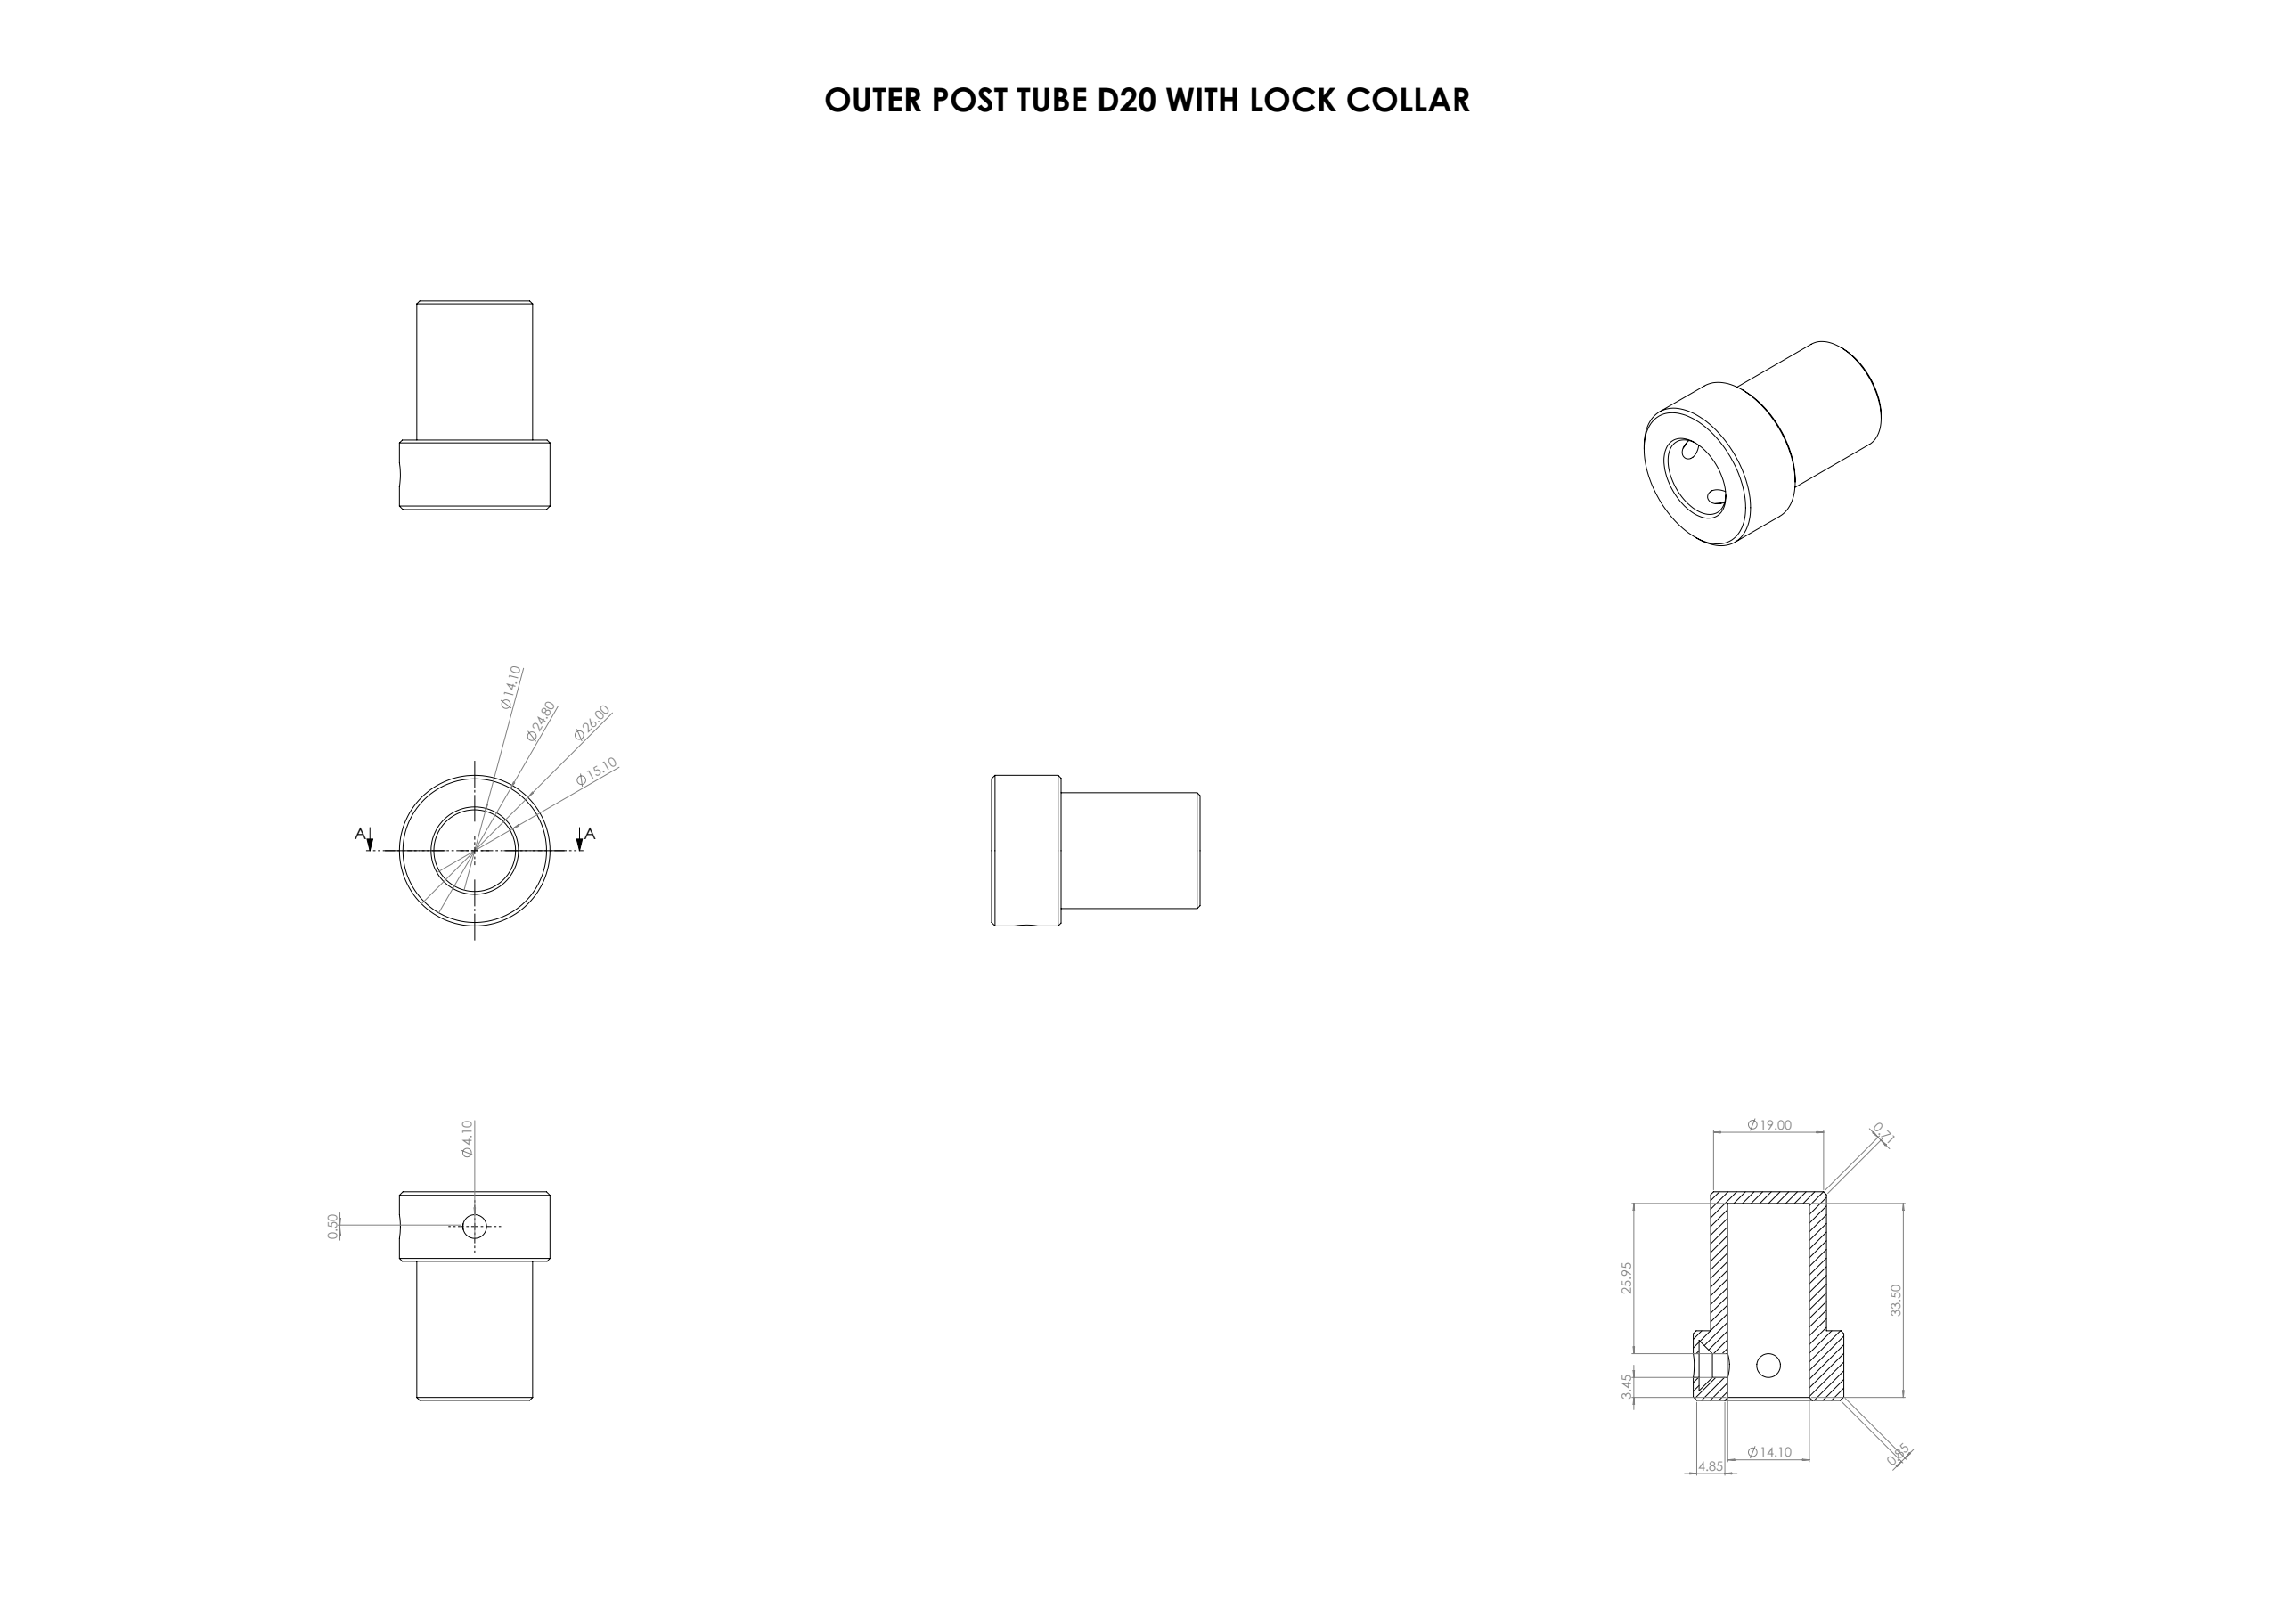
ISO-10303-21;
HEADER;
/* Generated by software containing ST-Developer
 * from STEP Tools, Inc. (www.steptools.com) 
 */

FILE_DESCRIPTION(
/* description */ (''),
/* implementation_level */ '2;1');

FILE_NAME(
/* name */ 
'02_Outer_Post_Tube_D20_with_Lock_Collar.step',
/* time_stamp */ '2026-10-20T10:06:23-07:00',
/* author */ (''),
/* organization */ (''),
/* preprocessor_version */ 'ST-DEVELOPER v20.2',
/* originating_system */ 'Autodesk Translation Framework v15.15.0.0',
/* authorisation */ '');

FILE_SCHEMA (('AUTOMOTIVE_DESIGN { 1 0 10303 214 3 1 1 }'));
ENDSEC;

DATA;
#10=MECHANICAL_DESIGN_GEOMETRIC_PRESENTATION_REPRESENTATION('',(#461),#38611);
#433=SHAPE_REPRESENTATION_RELATIONSHIP('SRR','None',#38669,#447);
#447=ADVANCED_BREP_SHAPE_REPRESENTATION('',(#475),#38598);
#461=STYLED_ITEM('',(#38871),#475);
#475=MANIFOLD_SOLID_BREP('Tube',#16235);
#516=B_SPLINE_CURVE_WITH_KNOTS('',3,(#22682,#22683,#22684,#22685,#22686,
#22687,#22688,#22689,#22690,#22691),.UNSPECIFIED.,.F.,.F.,(4,2,2,2,4),(0.024631319172959,
0.0777176003976506,0.155435200795301,0.233132476857833,0.310829752920366),
 .UNSPECIFIED.);
#517=B_SPLINE_CURVE_WITH_KNOTS('',3,(#22695,#22696,#22697,#22698,#22699,
#22700,#22701,#22702,#22703,#22704),.UNSPECIFIED.,.F.,.F.,(4,2,2,2,4),(0.932489258761097,
1.01018653482363,1.08788381088616,1.16560141128381,1.2186876925085),
 .UNSPECIFIED.);
#518=B_SPLINE_CURVE_WITH_KNOTS('',3,(#22707,#22708,#22709,#22710,#22711,
#22712,#22713,#22714,#22715,#22716),.UNSPECIFIED.,.F.,.F.,(4,2,2,2,4),(0.64629082501369,
0.699377106238382,0.777094706636032,0.854791982698564,0.932489258761097),
 .UNSPECIFIED.);
#519=B_SPLINE_CURVE_WITH_KNOTS('',3,(#22719,#22720,#22721,#22722,#22723,
#22724,#22725,#22726,#22727,#22728),.UNSPECIFIED.,.F.,.F.,(4,2,2,2,4),(0.310829752920366,
0.388527028982898,0.46622430504543,0.54394190544308,0.597028186667772),
 .UNSPECIFIED.);
#520=B_SPLINE_CURVE_WITH_KNOTS('',3,(#22741,#22742,#22743,#22744,#22745,
#22746,#22747,#22748,#22749,#22750,#22751,#22752,#22753,#22754,#22755,#22756,
#22757,#22758,#22759,#22760,#22761,#22762,#22763,#22764,#22765,#22766),
 .UNSPECIFIED.,.F.,.F.,(4,2,2,2,2,2,2,2,2,2,2,2,4),(0.,0.0773604855652864,
0.154720971130573,0.232079805418848,0.309438639707124,0.3867974739954,0.464156308283676,
0.541516793848962,0.618877279414249,0.696237764979535,0.773598250544821,
0.850957084833097,0.928315919121373),.UNSPECIFIED.);
#521=B_SPLINE_CURVE_WITH_KNOTS('',3,(#22767,#22768,#22769,#22770,#22771,
#22772,#22773,#22774,#22775,#22776),.UNSPECIFIED.,.F.,.F.,(4,2,2,2,4),(0.928315919121373,
1.00567475340965,1.08303358769792,1.16039407326321,1.2377545588285),
 .UNSPECIFIED.);
#522=B_SPLINE_CURVE_WITH_KNOTS('',3,(#22786,#22787,#22788,#22789,#22790,
#22791,#22792,#22793,#22794,#22795),.UNSPECIFIED.,.F.,.F.,(4,2,2,2,4),(0.,
0.0773604855652864,0.154720971130573,0.232079805418848,0.309438639707124),
 .UNSPECIFIED.);
#523=B_SPLINE_CURVE_WITH_KNOTS('',3,(#22797,#22798,#22799,#22800,#22801,
#22802,#22803,#22804,#22805,#22806),.UNSPECIFIED.,.F.,.F.,(4,2,2,2,4),(0.928315919121373,
1.00567475340965,1.08303358769792,1.16039407326321,1.2377545588285),
 .UNSPECIFIED.);
#524=B_SPLINE_CURVE_WITH_KNOTS('',3,(#22807,#22808,#22809,#22810,#22811,
#22812,#22813,#22814,#22815,#22816,#22817,#22818,#22819,#22820,#22821,#22822,
#22823,#22824),.UNSPECIFIED.,.F.,.F.,(4,2,2,2,2,2,2,2,4),(0.309438639707124,
0.3867974739954,0.464156308283676,0.541516793848962,0.618877279414249,0.696237764979535,
0.773598250544821,0.850957084833097,0.928315919121373),.UNSPECIFIED.);
#525=B_SPLINE_CURVE_WITH_KNOTS('',3,(#22834,#22835,#22836,#22837,#22838,
#22839,#22840,#22841,#22842,#22843),.UNSPECIFIED.,.F.,.F.,(4,2,2,2,4),(0.0246313191729586,
0.0777176003976506,0.155435200795301,0.233132476857833,0.310829752920366),
 .UNSPECIFIED.);
#526=B_SPLINE_CURVE_WITH_KNOTS('',3,(#22846,#22847,#22848,#22849,#22850,
#22851,#22852,#22853,#22854,#22855,#22856,#22857,#22858,#22859,#22860,#22861,
#22862,#22863),.UNSPECIFIED.,.F.,.F.,(4,2,2,2,2,2,2,2,4),(0.64629082501369,
0.699377106238382,0.777094706636033,0.854791982698565,0.932489258761097,
1.01018653482363,1.08788381088616,1.16560141128381,1.2186876925085),
 .UNSPECIFIED.);
#527=B_SPLINE_CURVE_WITH_KNOTS('',3,(#22864,#22865,#22866,#22867,#22868,
#22869,#22870,#22871,#22872,#22873),.UNSPECIFIED.,.F.,.F.,(4,2,2,2,4),(0.310829752920366,
0.388527028982898,0.46622430504543,0.543941905443081,0.597028186667773),
 .UNSPECIFIED.);
#888=CYLINDRICAL_SURFACE('',#16587,0.205);
#889=CYLINDRICAL_SURFACE('',#16595,0.205);
#890=CYLINDRICAL_SURFACE('',#16598,0.205);
#891=CYLINDRICAL_SURFACE('',#16601,0.205);
#892=CYLINDRICAL_SURFACE('',#16608,1.);
#893=CYLINDRICAL_SURFACE('',#16614,1.3);
#894=CYLINDRICAL_SURFACE('',#16622,0.705);
#1163=FACE_BOUND('',#2820,.T.);
#1164=FACE_BOUND('',#2825,.T.);
#1165=FACE_BOUND('',#2837,.T.);
#1166=FACE_BOUND('',#2840,.T.);
#1167=FACE_BOUND('',#2843,.T.);
#1168=FACE_BOUND('',#2846,.T.);
#1259=CIRCLE('',#16583,0.435);
#1260=CIRCLE('',#16584,0.205);
#1261=CIRCLE('',#16586,0.205);
#1262=CIRCLE('',#16588,0.205);
#1263=CIRCLE('',#16589,0.205);
#1264=CIRCLE('',#16591,0.435);
#1265=CIRCLE('',#16592,0.205);
#1266=CIRCLE('',#16594,0.205);
#1267=CIRCLE('',#16600,0.205);
#1268=CIRCLE('',#16602,0.205);
#1269=CIRCLE('',#16605,0.95);
#1270=CIRCLE('',#16607,1.);
#1271=CIRCLE('',#16609,1.);
#1272=CIRCLE('',#16611,1.25);
#1273=CIRCLE('',#16613,1.3);
#1274=CIRCLE('',#16615,1.3);
#1275=CIRCLE('',#16617,1.24);
#1276=CIRCLE('',#16619,0.755);
#1277=CIRCLE('',#16621,0.705);
#1278=CIRCLE('',#16623,0.705);
#1703=CONICAL_SURFACE('',#16585,0.2175,0.785398163397448);
#1704=CONICAL_SURFACE('',#16590,0.435,0.785398163397448);
#1705=CONICAL_SURFACE('',#16606,0.975,0.785398163397449);
#1706=CONICAL_SURFACE('',#16612,1.275,0.785398163397446);
#1707=CONICAL_SURFACE('',#16616,1.27,0.785398163397448);
#1708=CONICAL_SURFACE('',#16620,0.73,0.785398163397451);
#1898=FACE_OUTER_BOUND('',#2819,.T.);
#1899=FACE_OUTER_BOUND('',#2821,.T.);
#1900=FACE_OUTER_BOUND('',#2822,.T.);
#1901=FACE_OUTER_BOUND('',#2823,.T.);
#1902=FACE_OUTER_BOUND('',#2824,.T.);
#1903=FACE_OUTER_BOUND('',#2826,.T.);
#1904=FACE_OUTER_BOUND('',#2827,.T.);
#1905=FACE_OUTER_BOUND('',#2828,.T.);
#1906=FACE_OUTER_BOUND('',#2829,.T.);
#1907=FACE_OUTER_BOUND('',#2830,.T.);
#1908=FACE_OUTER_BOUND('',#2831,.T.);
#1909=FACE_OUTER_BOUND('',#2832,.T.);
#1910=FACE_OUTER_BOUND('',#2833,.T.);
#1911=FACE_OUTER_BOUND('',#2834,.T.);
#1912=FACE_OUTER_BOUND('',#2835,.T.);
#1913=FACE_OUTER_BOUND('',#2836,.T.);
#1914=FACE_OUTER_BOUND('',#2838,.T.);
#1915=FACE_OUTER_BOUND('',#2839,.T.);
#1916=FACE_OUTER_BOUND('',#2841,.T.);
#1917=FACE_OUTER_BOUND('',#2842,.T.);
#1918=FACE_OUTER_BOUND('',#2844,.T.);
#1919=FACE_OUTER_BOUND('',#2845,.T.);
#1920=FACE_OUTER_BOUND('',#2847,.T.);
#2819=EDGE_LOOP('',(#10609));
#2820=EDGE_LOOP('',(#10610));
#2821=EDGE_LOOP('',(#10611,#10612,#10613,#10614));
#2822=EDGE_LOOP('',(#10615,#10616,#10617,#10618,#10619,#10620,#10621,#10622,
#10623));
#2823=EDGE_LOOP('',(#10624,#10625,#10626,#10627));
#2824=EDGE_LOOP('',(#10628));
#2825=EDGE_LOOP('',(#10629));
#2826=EDGE_LOOP('',(#10630,#10631,#10632,#10633,#10634));
#2827=EDGE_LOOP('',(#10635,#10636));
#2828=EDGE_LOOP('',(#10637,#10638));
#2829=EDGE_LOOP('',(#10639,#10640,#10641,#10642,#10643,#10644));
#2830=EDGE_LOOP('',(#10645,#10646));
#2831=EDGE_LOOP('',(#10647,#10648,#10649,#10650,#10651,#10652,#10653,#10654));
#2832=EDGE_LOOP('',(#10655,#10656));
#2833=EDGE_LOOP('',(#10657));
#2834=EDGE_LOOP('',(#10658,#10659,#10660,#10661));
#2835=EDGE_LOOP('',(#10662,#10663,#10664,#10665));
#2836=EDGE_LOOP('',(#10666));
#2837=EDGE_LOOP('',(#10667));
#2838=EDGE_LOOP('',(#10668,#10669,#10670,#10671));
#2839=EDGE_LOOP('',(#10672,#10673,#10674,#10675,#10676,#10677,#10678,#10679,
#10680));
#2840=EDGE_LOOP('',(#10681,#10682));
#2841=EDGE_LOOP('',(#10683,#10684,#10685,#10686));
#2842=EDGE_LOOP('',(#10687));
#2843=EDGE_LOOP('',(#10688));
#2844=EDGE_LOOP('',(#10689,#10690,#10691,#10692));
#2845=EDGE_LOOP('',(#10693,#10694,#10695,#10696,#10697,#10698,#10699,#10700,
#10701,#10702,#10703,#10704));
#2846=EDGE_LOOP('',(#10705,#10706,#10707,#10708,#10709));
#2847=EDGE_LOOP('',(#10710));
#3889=LINE('',#22678,#5113);
#3890=LINE('',#22705,#5114);
#3891=LINE('',#22733,#5115);
#3892=LINE('',#22777,#5116);
#3893=LINE('',#22779,#5117);
#3894=LINE('',#22781,#5118);
#3895=LINE('',#22784,#5119);
#3896=LINE('',#22828,#5120);
#3897=LINE('',#22832,#5121);
#3898=LINE('',#22875,#5122);
#3899=LINE('',#22882,#5123);
#3900=LINE('',#22886,#5124);
#3901=LINE('',#22893,#5125);
#3902=LINE('',#22897,#5126);
#3903=LINE('',#22898,#5127);
#3904=LINE('',#22902,#5128);
#3905=LINE('',#22908,#5129);
#3906=LINE('',#22911,#5130);
#3907=LINE('',#22913,#5131);
#5113=VECTOR('',#18408,0.2175);
#5114=VECTOR('',#18413,0.205);
#5115=VECTOR('',#18420,0.435);
#5116=VECTOR('',#18429,0.205);
#5117=VECTOR('',#18432,1.);
#5118=VECTOR('',#18435,1.);
#5119=VECTOR('',#18438,0.205);
#5120=VECTOR('',#18441,1.);
#5121=VECTOR('',#18446,0.205);
#5122=VECTOR('',#18451,1.);
#5123=VECTOR('',#18460,0.975);
#5124=VECTOR('',#18465,1.);
#5125=VECTOR('',#18474,1.275);
#5126=VECTOR('',#18479,1.3);
#5127=VECTOR('',#18480,1.3);
#5128=VECTOR('',#18485,1.27);
#5129=VECTOR('',#18492,0.73);
#5130=VECTOR('',#18497,0.705);
#5131=VECTOR('',#18498,0.705);
#6277=VERTEX_POINT('',#22671);
#6278=VERTEX_POINT('',#22673);
#6279=VERTEX_POINT('',#22676);
#6280=VERTEX_POINT('',#22680);
#6281=VERTEX_POINT('',#22681);
#6282=VERTEX_POINT('',#22692);
#6283=VERTEX_POINT('',#22694);
#6284=VERTEX_POINT('',#22706);
#6285=VERTEX_POINT('',#22717);
#6286=VERTEX_POINT('',#22730);
#6287=VERTEX_POINT('',#22732);
#6288=VERTEX_POINT('',#22736);
#6289=VERTEX_POINT('',#22739);
#6290=VERTEX_POINT('',#22740);
#6291=VERTEX_POINT('',#22783);
#6292=VERTEX_POINT('',#22785);
#6293=VERTEX_POINT('',#22796);
#6294=VERTEX_POINT('',#22826);
#6295=VERTEX_POINT('',#22827);
#6296=VERTEX_POINT('',#22831);
#6297=VERTEX_POINT('',#22833);
#6298=VERTEX_POINT('',#22844);
#6299=VERTEX_POINT('',#22877);
#6300=VERTEX_POINT('',#22880);
#6301=VERTEX_POINT('',#22884);
#6302=VERTEX_POINT('',#22888);
#6303=VERTEX_POINT('',#22891);
#6304=VERTEX_POINT('',#22895);
#6305=VERTEX_POINT('',#22900);
#6306=VERTEX_POINT('',#22904);
#6307=VERTEX_POINT('',#22907);
#6308=VERTEX_POINT('',#22912);
#7920=EDGE_CURVE('',#6277,#6277,#1259,.T.);
#7921=EDGE_CURVE('',#6278,#6278,#1260,.T.);
#7922=EDGE_CURVE('',#6279,#6279,#1261,.T.);
#7923=EDGE_CURVE('',#6279,#6277,#3889,.T.);
#7924=EDGE_CURVE('',#6280,#6281,#516,.T.);
#7925=EDGE_CURVE('',#6282,#6280,#1262,.T.);
#7926=EDGE_CURVE('',#6283,#6282,#517,.T.);
#7927=EDGE_CURVE('',#6283,#6279,#3890,.T.);
#7928=EDGE_CURVE('',#6284,#6283,#518,.T.);
#7929=EDGE_CURVE('',#6285,#6284,#1263,.T.);
#7930=EDGE_CURVE('',#6281,#6285,#519,.T.);
#7931=EDGE_CURVE('',#6286,#6286,#1264,.T.);
#7932=EDGE_CURVE('',#6286,#6287,#3891,.T.);
#7933=EDGE_CURVE('',#6287,#6287,#1265,.T.);
#7934=EDGE_CURVE('',#6288,#6288,#1266,.T.);
#7935=EDGE_CURVE('',#6289,#6290,#520,.T.);
#7936=EDGE_CURVE('',#6290,#6289,#521,.T.);
#7937=EDGE_CURVE('',#6290,#6288,#3892,.T.);
#7938=EDGE_CURVE('',#6282,#6280,#3893,.T.);
#7939=EDGE_CURVE('',#6285,#6284,#3894,.T.);
#7940=EDGE_CURVE('',#6278,#6291,#3895,.T.);
#7941=EDGE_CURVE('',#6292,#6291,#522,.T.);
#7942=EDGE_CURVE('',#6293,#6292,#523,.T.);
#7943=EDGE_CURVE('',#6291,#6293,#524,.T.);
#7944=EDGE_CURVE('',#6294,#6295,#3896,.T.);
#7945=EDGE_CURVE('',#6295,#6294,#1267,.T.);
#7946=EDGE_CURVE('',#6287,#6296,#3897,.T.);
#7947=EDGE_CURVE('',#6297,#6296,#525,.T.);
#7948=EDGE_CURVE('',#6297,#6298,#1268,.T.);
#7949=EDGE_CURVE('',#6295,#6298,#526,.T.);
#7950=EDGE_CURVE('',#6296,#6294,#527,.T.);
#7951=EDGE_CURVE('',#6298,#6297,#3898,.T.);
#7952=EDGE_CURVE('',#6299,#6299,#1269,.T.);
#7953=EDGE_CURVE('',#6300,#6300,#1270,.T.);
#7954=EDGE_CURVE('',#6300,#6299,#3899,.T.);
#7955=EDGE_CURVE('',#6301,#6301,#1271,.T.);
#7956=EDGE_CURVE('',#6301,#6300,#3900,.T.);
#7957=EDGE_CURVE('',#6302,#6302,#1272,.T.);
#7958=EDGE_CURVE('',#6303,#6303,#1273,.T.);
#7959=EDGE_CURVE('',#6303,#6302,#3901,.T.);
#7960=EDGE_CURVE('',#6304,#6304,#1274,.T.);
#7961=EDGE_CURVE('',#6304,#6293,#3902,.T.);
#7962=EDGE_CURVE('',#6291,#6303,#3903,.T.);
#7963=EDGE_CURVE('',#6305,#6305,#1275,.T.);
#7964=EDGE_CURVE('',#6305,#6304,#3904,.T.);
#7965=EDGE_CURVE('',#6306,#6306,#1276,.T.);
#7966=EDGE_CURVE('',#6306,#6307,#3905,.T.);
#7967=EDGE_CURVE('',#6307,#6307,#1277,.T.);
#7968=EDGE_CURVE('',#6307,#6281,#3906,.T.);
#7969=EDGE_CURVE('',#6283,#6308,#3907,.T.);
#7970=EDGE_CURVE('',#6308,#6308,#1278,.T.);
#10609=ORIENTED_EDGE('',*,*,#7920,.F.);
#10610=ORIENTED_EDGE('',*,*,#7921,.F.);
#10611=ORIENTED_EDGE('',*,*,#7922,.F.);
#10612=ORIENTED_EDGE('',*,*,#7923,.T.);
#10613=ORIENTED_EDGE('',*,*,#7920,.T.);
#10614=ORIENTED_EDGE('',*,*,#7923,.F.);
#10615=ORIENTED_EDGE('',*,*,#7924,.F.);
#10616=ORIENTED_EDGE('',*,*,#7925,.F.);
#10617=ORIENTED_EDGE('',*,*,#7926,.F.);
#10618=ORIENTED_EDGE('',*,*,#7927,.T.);
#10619=ORIENTED_EDGE('',*,*,#7922,.T.);
#10620=ORIENTED_EDGE('',*,*,#7927,.F.);
#10621=ORIENTED_EDGE('',*,*,#7928,.F.);
#10622=ORIENTED_EDGE('',*,*,#7929,.F.);
#10623=ORIENTED_EDGE('',*,*,#7930,.F.);
#10624=ORIENTED_EDGE('',*,*,#7931,.F.);
#10625=ORIENTED_EDGE('',*,*,#7932,.T.);
#10626=ORIENTED_EDGE('',*,*,#7933,.F.);
#10627=ORIENTED_EDGE('',*,*,#7932,.F.);
#10628=ORIENTED_EDGE('',*,*,#7931,.T.);
#10629=ORIENTED_EDGE('',*,*,#7934,.F.);
#10630=ORIENTED_EDGE('',*,*,#7935,.F.);
#10631=ORIENTED_EDGE('',*,*,#7936,.F.);
#10632=ORIENTED_EDGE('',*,*,#7937,.T.);
#10633=ORIENTED_EDGE('',*,*,#7934,.T.);
#10634=ORIENTED_EDGE('',*,*,#7937,.F.);
#10635=ORIENTED_EDGE('',*,*,#7938,.F.);
#10636=ORIENTED_EDGE('',*,*,#7925,.T.);
#10637=ORIENTED_EDGE('',*,*,#7939,.F.);
#10638=ORIENTED_EDGE('',*,*,#7929,.T.);
#10639=ORIENTED_EDGE('',*,*,#7921,.T.);
#10640=ORIENTED_EDGE('',*,*,#7940,.T.);
#10641=ORIENTED_EDGE('',*,*,#7941,.F.);
#10642=ORIENTED_EDGE('',*,*,#7942,.F.);
#10643=ORIENTED_EDGE('',*,*,#7943,.F.);
#10644=ORIENTED_EDGE('',*,*,#7940,.F.);
#10645=ORIENTED_EDGE('',*,*,#7944,.F.);
#10646=ORIENTED_EDGE('',*,*,#7945,.F.);
#10647=ORIENTED_EDGE('',*,*,#7933,.T.);
#10648=ORIENTED_EDGE('',*,*,#7946,.T.);
#10649=ORIENTED_EDGE('',*,*,#7947,.F.);
#10650=ORIENTED_EDGE('',*,*,#7948,.T.);
#10651=ORIENTED_EDGE('',*,*,#7949,.F.);
#10652=ORIENTED_EDGE('',*,*,#7945,.T.);
#10653=ORIENTED_EDGE('',*,*,#7950,.F.);
#10654=ORIENTED_EDGE('',*,*,#7946,.F.);
#10655=ORIENTED_EDGE('',*,*,#7951,.F.);
#10656=ORIENTED_EDGE('',*,*,#7948,.F.);
#10657=ORIENTED_EDGE('',*,*,#7952,.F.);
#10658=ORIENTED_EDGE('',*,*,#7953,.F.);
#10659=ORIENTED_EDGE('',*,*,#7954,.T.);
#10660=ORIENTED_EDGE('',*,*,#7952,.T.);
#10661=ORIENTED_EDGE('',*,*,#7954,.F.);
#10662=ORIENTED_EDGE('',*,*,#7955,.F.);
#10663=ORIENTED_EDGE('',*,*,#7956,.T.);
#10664=ORIENTED_EDGE('',*,*,#7953,.T.);
#10665=ORIENTED_EDGE('',*,*,#7956,.F.);
#10666=ORIENTED_EDGE('',*,*,#7957,.F.);
#10667=ORIENTED_EDGE('',*,*,#7955,.T.);
#10668=ORIENTED_EDGE('',*,*,#7958,.F.);
#10669=ORIENTED_EDGE('',*,*,#7959,.T.);
#10670=ORIENTED_EDGE('',*,*,#7957,.T.);
#10671=ORIENTED_EDGE('',*,*,#7959,.F.);
#10672=ORIENTED_EDGE('',*,*,#7960,.F.);
#10673=ORIENTED_EDGE('',*,*,#7961,.T.);
#10674=ORIENTED_EDGE('',*,*,#7942,.T.);
#10675=ORIENTED_EDGE('',*,*,#7941,.T.);
#10676=ORIENTED_EDGE('',*,*,#7962,.T.);
#10677=ORIENTED_EDGE('',*,*,#7958,.T.);
#10678=ORIENTED_EDGE('',*,*,#7962,.F.);
#10679=ORIENTED_EDGE('',*,*,#7943,.T.);
#10680=ORIENTED_EDGE('',*,*,#7961,.F.);
#10681=ORIENTED_EDGE('',*,*,#7935,.T.);
#10682=ORIENTED_EDGE('',*,*,#7936,.T.);
#10683=ORIENTED_EDGE('',*,*,#7963,.F.);
#10684=ORIENTED_EDGE('',*,*,#7964,.T.);
#10685=ORIENTED_EDGE('',*,*,#7960,.T.);
#10686=ORIENTED_EDGE('',*,*,#7964,.F.);
#10687=ORIENTED_EDGE('',*,*,#7963,.T.);
#10688=ORIENTED_EDGE('',*,*,#7965,.F.);
#10689=ORIENTED_EDGE('',*,*,#7965,.T.);
#10690=ORIENTED_EDGE('',*,*,#7966,.T.);
#10691=ORIENTED_EDGE('',*,*,#7967,.F.);
#10692=ORIENTED_EDGE('',*,*,#7966,.F.);
#10693=ORIENTED_EDGE('',*,*,#7967,.T.);
#10694=ORIENTED_EDGE('',*,*,#7968,.T.);
#10695=ORIENTED_EDGE('',*,*,#7930,.T.);
#10696=ORIENTED_EDGE('',*,*,#7939,.T.);
#10697=ORIENTED_EDGE('',*,*,#7928,.T.);
#10698=ORIENTED_EDGE('',*,*,#7969,.T.);
#10699=ORIENTED_EDGE('',*,*,#7970,.F.);
#10700=ORIENTED_EDGE('',*,*,#7969,.F.);
#10701=ORIENTED_EDGE('',*,*,#7926,.T.);
#10702=ORIENTED_EDGE('',*,*,#7938,.T.);
#10703=ORIENTED_EDGE('',*,*,#7924,.T.);
#10704=ORIENTED_EDGE('',*,*,#7968,.F.);
#10705=ORIENTED_EDGE('',*,*,#7949,.T.);
#10706=ORIENTED_EDGE('',*,*,#7951,.T.);
#10707=ORIENTED_EDGE('',*,*,#7947,.T.);
#10708=ORIENTED_EDGE('',*,*,#7950,.T.);
#10709=ORIENTED_EDGE('',*,*,#7944,.T.);
#10710=ORIENTED_EDGE('',*,*,#7970,.T.);
#14886=PLANE('',#16582);
#14887=PLANE('',#16593);
#14888=PLANE('',#16596);
#14889=PLANE('',#16597);
#14890=PLANE('',#16599);
#14891=PLANE('',#16603);
#14892=PLANE('',#16604);
#14893=PLANE('',#16610);
#14894=PLANE('',#16618);
#14895=PLANE('',#16624);
#15441=ADVANCED_FACE('',(#1898,#1163),#14886,.F.);
#15442=ADVANCED_FACE('',(#1899),#1703,.F.);
#15443=ADVANCED_FACE('',(#1900),#888,.F.);
#15444=ADVANCED_FACE('',(#1901),#1704,.F.);
#15445=ADVANCED_FACE('',(#1902,#1164),#14887,.F.);
#15446=ADVANCED_FACE('',(#1903),#889,.F.);
#15447=ADVANCED_FACE('',(#1904),#14888,.F.);
#15448=ADVANCED_FACE('',(#1905),#14889,.F.);
#15449=ADVANCED_FACE('',(#1906),#890,.F.);
#15450=ADVANCED_FACE('',(#1907),#14890,.F.);
#15451=ADVANCED_FACE('',(#1908),#891,.F.);
#15452=ADVANCED_FACE('',(#1909),#14891,.F.);
#15453=ADVANCED_FACE('',(#1910),#14892,.T.);
#15454=ADVANCED_FACE('',(#1911),#1705,.T.);
#15455=ADVANCED_FACE('',(#1912),#892,.T.);
#15456=ADVANCED_FACE('',(#1913,#1165),#14893,.T.);
#15457=ADVANCED_FACE('',(#1914),#1706,.T.);
#15458=ADVANCED_FACE('',(#1915,#1166),#893,.T.);
#15459=ADVANCED_FACE('',(#1916),#1707,.T.);
#15460=ADVANCED_FACE('',(#1917,#1167),#14894,.T.);
#15461=ADVANCED_FACE('',(#1918),#1708,.F.);
#15462=ADVANCED_FACE('',(#1919,#1168),#894,.F.);
#15463=ADVANCED_FACE('',(#1920),#14895,.T.);
#16235=CLOSED_SHELL('',(#15441,#15442,#15443,#15444,#15445,#15446,#15447,
#15448,#15449,#15450,#15451,#15452,#15453,#15454,#15455,#15456,#15457,#15458,
#15459,#15460,#15461,#15462,#15463));
#16581=AXIS2_PLACEMENT_3D('',#22669,#18396,#18397);
#16582=AXIS2_PLACEMENT_3D('',#22670,#18398,#18399);
#16583=AXIS2_PLACEMENT_3D('',#22672,#18400,#18401);
#16584=AXIS2_PLACEMENT_3D('',#22674,#18402,#18403);
#16585=AXIS2_PLACEMENT_3D('',#22675,#18404,#18405);
#16586=AXIS2_PLACEMENT_3D('',#22677,#18406,#18407);
#16587=AXIS2_PLACEMENT_3D('',#22679,#18409,#18410);
#16588=AXIS2_PLACEMENT_3D('',#22693,#18411,#18412);
#16589=AXIS2_PLACEMENT_3D('',#22718,#18414,#18415);
#16590=AXIS2_PLACEMENT_3D('',#22729,#18416,#18417);
#16591=AXIS2_PLACEMENT_3D('',#22731,#18418,#18419);
#16592=AXIS2_PLACEMENT_3D('',#22734,#18421,#18422);
#16593=AXIS2_PLACEMENT_3D('',#22735,#18423,#18424);
#16594=AXIS2_PLACEMENT_3D('',#22737,#18425,#18426);
#16595=AXIS2_PLACEMENT_3D('',#22738,#18427,#18428);
#16596=AXIS2_PLACEMENT_3D('',#22778,#18430,#18431);
#16597=AXIS2_PLACEMENT_3D('',#22780,#18433,#18434);
#16598=AXIS2_PLACEMENT_3D('',#22782,#18436,#18437);
#16599=AXIS2_PLACEMENT_3D('',#22825,#18439,#18440);
#16600=AXIS2_PLACEMENT_3D('',#22829,#18442,#18443);
#16601=AXIS2_PLACEMENT_3D('',#22830,#18444,#18445);
#16602=AXIS2_PLACEMENT_3D('',#22845,#18447,#18448);
#16603=AXIS2_PLACEMENT_3D('',#22874,#18449,#18450);
#16604=AXIS2_PLACEMENT_3D('',#22876,#18452,#18453);
#16605=AXIS2_PLACEMENT_3D('',#22878,#18454,#18455);
#16606=AXIS2_PLACEMENT_3D('',#22879,#18456,#18457);
#16607=AXIS2_PLACEMENT_3D('',#22881,#18458,#18459);
#16608=AXIS2_PLACEMENT_3D('',#22883,#18461,#18462);
#16609=AXIS2_PLACEMENT_3D('',#22885,#18463,#18464);
#16610=AXIS2_PLACEMENT_3D('',#22887,#18466,#18467);
#16611=AXIS2_PLACEMENT_3D('',#22889,#18468,#18469);
#16612=AXIS2_PLACEMENT_3D('',#22890,#18470,#18471);
#16613=AXIS2_PLACEMENT_3D('',#22892,#18472,#18473);
#16614=AXIS2_PLACEMENT_3D('',#22894,#18475,#18476);
#16615=AXIS2_PLACEMENT_3D('',#22896,#18477,#18478);
#16616=AXIS2_PLACEMENT_3D('',#22899,#18481,#18482);
#16617=AXIS2_PLACEMENT_3D('',#22901,#18483,#18484);
#16618=AXIS2_PLACEMENT_3D('',#22903,#18486,#18487);
#16619=AXIS2_PLACEMENT_3D('',#22905,#18488,#18489);
#16620=AXIS2_PLACEMENT_3D('',#22906,#18490,#18491);
#16621=AXIS2_PLACEMENT_3D('',#22909,#18493,#18494);
#16622=AXIS2_PLACEMENT_3D('',#22910,#18495,#18496);
#16623=AXIS2_PLACEMENT_3D('',#22914,#18499,#18500);
#16624=AXIS2_PLACEMENT_3D('',#22915,#18501,#18502);
#18396=DIRECTION('axis',(0.,0.,1.));
#18397=DIRECTION('refdir',(1.,0.,0.));
#18398=DIRECTION('center_axis',(-1.,0.,0.));
#18399=DIRECTION('ref_axis',(0.,0.,1.));
#18400=DIRECTION('center_axis',(-1.,0.,0.));
#18401=DIRECTION('ref_axis',(0.,0.,1.));
#18402=DIRECTION('center_axis',(1.,0.,0.));
#18403=DIRECTION('ref_axis',(0.,0.,1.));
#18404=DIRECTION('center_axis',(-1.,0.,0.));
#18405=DIRECTION('ref_axis',(0.,0.,1.));
#18406=DIRECTION('center_axis',(-1.,0.,0.));
#18407=DIRECTION('ref_axis',(0.,0.,1.));
#18408=DIRECTION('',(-0.707106781186547,-8.65956056235493E-17,-0.707106781186548));
#18409=DIRECTION('center_axis',(-1.,0.,0.));
#18410=DIRECTION('ref_axis',(0.,0.,1.));
#18411=DIRECTION('center_axis',(-1.,0.,0.));
#18412=DIRECTION('ref_axis',(0.,0.,1.));
#18413=DIRECTION('',(-1.,0.,0.));
#18414=DIRECTION('center_axis',(-1.,0.,0.));
#18415=DIRECTION('ref_axis',(0.,0.,1.));
#18416=DIRECTION('center_axis',(0.,-1.,0.));
#18417=DIRECTION('ref_axis',(0.,0.,1.));
#18418=DIRECTION('center_axis',(0.,1.,0.));
#18419=DIRECTION('ref_axis',(1.,0.,0.));
#18420=DIRECTION('',(8.65956056235493E-17,0.707106781186547,0.707106781186548));
#18421=DIRECTION('center_axis',(0.,-1.,0.));
#18422=DIRECTION('ref_axis',(0.,0.,1.));
#18423=DIRECTION('center_axis',(0.,-1.,0.));
#18424=DIRECTION('ref_axis',(0.,0.,-1.));
#18425=DIRECTION('center_axis',(0.,1.,0.));
#18426=DIRECTION('ref_axis',(0.,0.,1.));
#18427=DIRECTION('center_axis',(0.,1.,0.));
#18428=DIRECTION('ref_axis',(0.,0.,1.));
#18429=DIRECTION('',(0.,1.,0.));
#18430=DIRECTION('center_axis',(1.,0.,0.));
#18431=DIRECTION('ref_axis',(0.,0.,-1.));
#18432=DIRECTION('',(0.,0.,1.));
#18433=DIRECTION('center_axis',(1.,0.,0.));
#18434=DIRECTION('ref_axis',(0.,0.,-1.));
#18435=DIRECTION('',(0.,0.,-1.));
#18436=DIRECTION('center_axis',(-1.,0.,0.));
#18437=DIRECTION('ref_axis',(0.,0.,1.));
#18438=DIRECTION('',(-1.,0.,0.));
#18439=DIRECTION('center_axis',(0.,1.,0.));
#18440=DIRECTION('ref_axis',(0.,0.,1.));
#18441=DIRECTION('',(0.,0.,1.));
#18442=DIRECTION('center_axis',(0.,1.,0.));
#18443=DIRECTION('ref_axis',(1.,0.,0.));
#18444=DIRECTION('center_axis',(0.,1.,0.));
#18445=DIRECTION('ref_axis',(0.,0.,1.));
#18446=DIRECTION('',(0.,1.,0.));
#18447=DIRECTION('center_axis',(0.,1.,0.));
#18448=DIRECTION('ref_axis',(1.,0.,0.));
#18449=DIRECTION('center_axis',(0.,1.,0.));
#18450=DIRECTION('ref_axis',(0.,0.,1.));
#18451=DIRECTION('',(0.,0.,-1.));
#18452=DIRECTION('center_axis',(0.,0.,-1.));
#18453=DIRECTION('ref_axis',(-1.,0.,0.));
#18454=DIRECTION('center_axis',(0.,0.,1.));
#18455=DIRECTION('ref_axis',(1.,0.,0.));
#18456=DIRECTION('center_axis',(0.,0.,1.));
#18457=DIRECTION('ref_axis',(1.,0.,0.));
#18458=DIRECTION('center_axis',(0.,0.,1.));
#18459=DIRECTION('ref_axis',(1.,0.,0.));
#18460=DIRECTION('',(0.707106781186548,8.65956056235494E-17,-0.707106781186547));
#18461=DIRECTION('center_axis',(0.,0.,1.));
#18462=DIRECTION('ref_axis',(1.,0.,0.));
#18463=DIRECTION('center_axis',(0.,0.,1.));
#18464=DIRECTION('ref_axis',(1.,0.,0.));
#18465=DIRECTION('',(0.,0.,-1.));
#18466=DIRECTION('center_axis',(0.,0.,-1.));
#18467=DIRECTION('ref_axis',(-1.,0.,0.));
#18468=DIRECTION('center_axis',(0.,0.,1.));
#18469=DIRECTION('ref_axis',(1.,0.,0.));
#18470=DIRECTION('center_axis',(0.,0.,1.));
#18471=DIRECTION('ref_axis',(1.,0.,0.));
#18472=DIRECTION('center_axis',(0.,0.,1.));
#18473=DIRECTION('ref_axis',(1.,0.,0.));
#18474=DIRECTION('',(0.707106781186546,8.65956056235491E-17,-0.707106781186549));
#18475=DIRECTION('center_axis',(0.,0.,1.));
#18476=DIRECTION('ref_axis',(1.,0.,0.));
#18477=DIRECTION('center_axis',(0.,0.,1.));
#18478=DIRECTION('ref_axis',(1.,0.,0.));
#18479=DIRECTION('',(0.,0.,-1.));
#18480=DIRECTION('',(0.,0.,-1.));
#18481=DIRECTION('center_axis',(0.,0.,-1.));
#18482=DIRECTION('ref_axis',(1.,0.,0.));
#18483=DIRECTION('center_axis',(0.,0.,1.));
#18484=DIRECTION('ref_axis',(1.,0.,0.));
#18485=DIRECTION('',(-0.707106781186547,-8.65956056235493E-17,-0.707106781186547));
#18486=DIRECTION('center_axis',(0.,0.,1.));
#18487=DIRECTION('ref_axis',(1.,0.,0.));
#18488=DIRECTION('center_axis',(0.,0.,1.));
#18489=DIRECTION('ref_axis',(1.,0.,0.));
#18490=DIRECTION('center_axis',(0.,0.,1.));
#18491=DIRECTION('ref_axis',(1.,0.,0.));
#18492=DIRECTION('',(0.707106781186549,8.65956056235495E-17,-0.707106781186546));
#18493=DIRECTION('center_axis',(0.,0.,1.));
#18494=DIRECTION('ref_axis',(1.,0.,0.));
#18495=DIRECTION('center_axis',(0.,0.,1.));
#18496=DIRECTION('ref_axis',(1.,0.,0.));
#18497=DIRECTION('',(0.,0.,-1.));
#18498=DIRECTION('',(0.,0.,-1.));
#18499=DIRECTION('center_axis',(0.,0.,1.));
#18500=DIRECTION('ref_axis',(1.,0.,0.));
#18501=DIRECTION('center_axis',(0.,0.,1.));
#18502=DIRECTION('ref_axis',(1.,0.,0.));
#22669=CARTESIAN_POINT('',(0.,0.,0.));
#22670=CARTESIAN_POINT('Origin',(-1.2,0.,3.4));
#22671=CARTESIAN_POINT('',(-1.2,-5.32721357629099E-17,2.965));
#22672=CARTESIAN_POINT('Origin',(-1.2,0.,3.4));
#22673=CARTESIAN_POINT('',(-1.2,2.51052593825207E-17,3.195));
#22674=CARTESIAN_POINT('Origin',(-1.2,0.,3.4));
#22675=CARTESIAN_POINT('Origin',(-0.9825,0.,3.4));
#22676=CARTESIAN_POINT('',(-0.97,-2.51052593825207E-17,3.195));
#22677=CARTESIAN_POINT('Origin',(-0.97,0.,3.4));
#22678=CARTESIAN_POINT('',(-0.9825,-2.66360678814549E-17,3.1825));
#22679=CARTESIAN_POINT('Origin',(-1.0025,0.,3.4));
#22680=CARTESIAN_POINT('',(-0.675,-0.203469899493758,3.425));
#22681=CARTESIAN_POINT('',(-0.705,-4.31687996699442E-17,3.605));
#22682=CARTESIAN_POINT('Ctrl Pts',(-0.675,-0.203469899493758,3.425));
#22683=CARTESIAN_POINT('Ctrl Pts',(-0.675671543655374,-0.201242091014444,
3.44313167869509));
#22684=CARTESIAN_POINT('Ctrl Pts',(-0.677111481787171,-0.196469587434997,
3.46142442095761));
#22685=CARTESIAN_POINT('Ctrl Pts',(-0.682029730751166,-0.178826374035794,
3.50388715643587));
#22686=CARTESIAN_POINT('Ctrl Pts',(-0.68612968485916,-0.16307623613103,
3.52683754415545));
#22687=CARTESIAN_POINT('Ctrl Pts',(-0.693742502155627,-0.126842282640148,
3.56307149764634));
#22688=CARTESIAN_POINT('Ctrl Pts',(-0.697765433634744,-0.103889959828094,
3.57882531009039));
#22689=CARTESIAN_POINT('Ctrl Pts',(-0.703431290629093,-0.0534241842031802,
3.59979357492158));
#22690=CARTESIAN_POINT('Ctrl Pts',(-0.705,-0.0258990920208441,3.605));
#22691=CARTESIAN_POINT('Ctrl Pts',(-0.705,-2.42861286636753E-17,3.605));
#22692=CARTESIAN_POINT('',(-0.675,-0.203469899493758,3.375));
#22693=CARTESIAN_POINT('Origin',(-0.675,0.,3.4));
#22694=CARTESIAN_POINT('',(-0.705,4.79460506850772E-18,3.195));
#22695=CARTESIAN_POINT('Ctrl Pts',(-0.705,3.46944695195361E-17,3.195));
#22696=CARTESIAN_POINT('Ctrl Pts',(-0.705,-0.0258990920208441,3.195));
#22697=CARTESIAN_POINT('Ctrl Pts',(-0.703431290629093,-0.0534241842031802,
3.20020642507842));
#22698=CARTESIAN_POINT('Ctrl Pts',(-0.697765433634744,-0.103889959828094,
3.22117468990961));
#22699=CARTESIAN_POINT('Ctrl Pts',(-0.693742502155627,-0.126842282640148,
3.23692850235366));
#22700=CARTESIAN_POINT('Ctrl Pts',(-0.68612968485916,-0.16307623613103,
3.27316245584455));
#22701=CARTESIAN_POINT('Ctrl Pts',(-0.682029730751167,-0.178826374035794,
3.29611284356413));
#22702=CARTESIAN_POINT('Ctrl Pts',(-0.677111481787171,-0.196469587434997,
3.33857557904239));
#22703=CARTESIAN_POINT('Ctrl Pts',(-0.675671543655374,-0.201242091014444,
3.35686832130491));
#22704=CARTESIAN_POINT('Ctrl Pts',(-0.675,-0.203469899493758,3.375));
#22705=CARTESIAN_POINT('',(-1.0025,-2.51052593825207E-17,3.195));
#22706=CARTESIAN_POINT('',(-0.675,0.203469899493758,3.375));
#22707=CARTESIAN_POINT('Ctrl Pts',(-0.675,0.203469899493758,3.375));
#22708=CARTESIAN_POINT('Ctrl Pts',(-0.675671543655374,0.201242091014444,
3.35686832130491));
#22709=CARTESIAN_POINT('Ctrl Pts',(-0.677111481787171,0.196469587434997,
3.33857557904239));
#22710=CARTESIAN_POINT('Ctrl Pts',(-0.682029730751166,0.178826374035794,
3.29611284356413));
#22711=CARTESIAN_POINT('Ctrl Pts',(-0.68612968485916,0.16307623613103,3.27316245584455));
#22712=CARTESIAN_POINT('Ctrl Pts',(-0.693742502155627,0.126842282640148,
3.23692850235366));
#22713=CARTESIAN_POINT('Ctrl Pts',(-0.697765433634744,0.103889959828094,
3.22117468990961));
#22714=CARTESIAN_POINT('Ctrl Pts',(-0.703431290629093,0.0534241842031802,
3.20020642507842));
#22715=CARTESIAN_POINT('Ctrl Pts',(-0.705,0.025899092020844,3.195));
#22716=CARTESIAN_POINT('Ctrl Pts',(-0.705,-4.16333634234434E-17,3.195));
#22717=CARTESIAN_POINT('',(-0.675,0.203469899493758,3.425));
#22718=CARTESIAN_POINT('Origin',(-0.675,0.,3.4));
#22719=CARTESIAN_POINT('Ctrl Pts',(-0.705,0.,3.605));
#22720=CARTESIAN_POINT('Ctrl Pts',(-0.705,0.025899092020844,3.605));
#22721=CARTESIAN_POINT('Ctrl Pts',(-0.703431290629093,0.0534241842031802,
3.59979357492158));
#22722=CARTESIAN_POINT('Ctrl Pts',(-0.697765433634744,0.103889959828094,
3.57882531009039));
#22723=CARTESIAN_POINT('Ctrl Pts',(-0.693742502155627,0.126842282640148,
3.56307149764634));
#22724=CARTESIAN_POINT('Ctrl Pts',(-0.68612968485916,0.16307623613103,3.52683754415545));
#22725=CARTESIAN_POINT('Ctrl Pts',(-0.682029730751166,0.178826374035794,
3.50388715643587));
#22726=CARTESIAN_POINT('Ctrl Pts',(-0.67711148178717,0.196469587434997,
3.46142442095761));
#22727=CARTESIAN_POINT('Ctrl Pts',(-0.675671543655374,0.201242091014444,
3.44313167869509));
#22728=CARTESIAN_POINT('Ctrl Pts',(-0.675,0.203469899493758,3.425));
#22729=CARTESIAN_POINT('Origin',(0.,-1.2,3.4));
#22730=CARTESIAN_POINT('',(-5.32721357629099E-17,-1.2,2.965));
#22731=CARTESIAN_POINT('Origin',(0.,-1.2,3.4));
#22732=CARTESIAN_POINT('',(2.51052593825207E-17,-0.97,3.195));
#22733=CARTESIAN_POINT('',(-5.32721357629099E-17,-1.2,2.965));
#22734=CARTESIAN_POINT('Origin',(0.,-0.97,3.4));
#22735=CARTESIAN_POINT('Origin',(0.,-1.2,3.835));
#22736=CARTESIAN_POINT('',(-2.51052593825207E-17,-1.2,3.195));
#22737=CARTESIAN_POINT('Origin',(0.,-1.2,3.4));
#22738=CARTESIAN_POINT('Origin',(0.,-1.0025,3.4));
#22739=CARTESIAN_POINT('',(-0.205,-1.28373478569368,3.4));
#22740=CARTESIAN_POINT('',(-2.51052593825207E-17,-1.3,3.195));
#22741=CARTESIAN_POINT('Ctrl Pts',(-0.205,-1.28373478569368,3.4));
#22742=CARTESIAN_POINT('Ctrl Pts',(-0.205,-1.28373478569368,3.42578682852176));
#22743=CARTESIAN_POINT('Ctrl Pts',(-0.199837668299145,-1.28459209201807,
3.45326250834418));
#22744=CARTESIAN_POINT('Ctrl Pts',(-0.178903418830812,-1.2876744550022,
3.50375720035387));
#22745=CARTESIAN_POINT('Ctrl Pts',(-0.163133809500307,-1.28985344916615,
3.52677997078618));
#22746=CARTESIAN_POINT('Ctrl Pts',(-0.12678035877662,-1.29393248914849,
3.56313342150986));
#22747=CARTESIAN_POINT('Ctrl Pts',(-0.103757421316811,-1.29609960028466,
3.57890333519745));
#22748=CARTESIAN_POINT('Ctrl Pts',(-0.0532621572488602,-1.29915469398922,
3.59983780588318));
#22749=CARTESIAN_POINT('Ctrl Pts',(-0.0257862780960919,-1.3,3.605));
#22750=CARTESIAN_POINT('Ctrl Pts',(0.0257862780960919,-1.3,3.605));
#22751=CARTESIAN_POINT('Ctrl Pts',(0.0532621572488602,-1.29915469398922,
3.59983780588318));
#22752=CARTESIAN_POINT('Ctrl Pts',(0.103757421316811,-1.29609960028466,
3.57890333519745));
#22753=CARTESIAN_POINT('Ctrl Pts',(0.12678035877662,-1.29393248914849,3.56313342150986));
#22754=CARTESIAN_POINT('Ctrl Pts',(0.163133809500307,-1.28985344916615,
3.52677997078618));
#22755=CARTESIAN_POINT('Ctrl Pts',(0.178903418830811,-1.2876744550022,3.50375720035387));
#22756=CARTESIAN_POINT('Ctrl Pts',(0.199837668299145,-1.28459209201807,
3.45326250834418));
#22757=CARTESIAN_POINT('Ctrl Pts',(0.205,-1.28373478569368,3.42578682852176));
#22758=CARTESIAN_POINT('Ctrl Pts',(0.205,-1.28373478569368,3.37421317147824));
#22759=CARTESIAN_POINT('Ctrl Pts',(0.199837668299145,-1.28459209201807,
3.34673749165582));
#22760=CARTESIAN_POINT('Ctrl Pts',(0.178903418830812,-1.2876744550022,3.29624279964613));
#22761=CARTESIAN_POINT('Ctrl Pts',(0.163133809500307,-1.28985344916615,
3.27322002921382));
#22762=CARTESIAN_POINT('Ctrl Pts',(0.12678035877662,-1.29393248914849,3.23686657849014));
#22763=CARTESIAN_POINT('Ctrl Pts',(0.103757421316811,-1.29609960028466,
3.22109666480255));
#22764=CARTESIAN_POINT('Ctrl Pts',(0.0532621572488603,-1.29915469398922,
3.20016219411682));
#22765=CARTESIAN_POINT('Ctrl Pts',(0.025786278096092,-1.3,3.195));
#22766=CARTESIAN_POINT('Ctrl Pts',(5.55111512312578E-17,-1.3,3.195));
#22767=CARTESIAN_POINT('Ctrl Pts',(3.81639164714898E-17,-1.3,3.195));
#22768=CARTESIAN_POINT('Ctrl Pts',(-0.0257862780960919,-1.3,3.195));
#22769=CARTESIAN_POINT('Ctrl Pts',(-0.0532621572488602,-1.29915469398922,
3.20016219411682));
#22770=CARTESIAN_POINT('Ctrl Pts',(-0.103757421316811,-1.29609960028466,
3.22109666480255));
#22771=CARTESIAN_POINT('Ctrl Pts',(-0.12678035877662,-1.29393248914849,
3.23686657849014));
#22772=CARTESIAN_POINT('Ctrl Pts',(-0.163133809500307,-1.28985344916615,
3.27322002921382));
#22773=CARTESIAN_POINT('Ctrl Pts',(-0.178903418830812,-1.2876744550022,
3.29624279964613));
#22774=CARTESIAN_POINT('Ctrl Pts',(-0.199837668299145,-1.28459209201807,
3.34673749165582));
#22775=CARTESIAN_POINT('Ctrl Pts',(-0.205,-1.28373478569368,3.37421317147824));
#22776=CARTESIAN_POINT('Ctrl Pts',(-0.205,-1.28373478569368,3.4));
#22777=CARTESIAN_POINT('',(-2.51052593825207E-17,-1.0025,3.195));
#22778=CARTESIAN_POINT('Origin',(-0.675,0.,3.605));
#22779=CARTESIAN_POINT('',(-0.675,-0.203469899493758,2.275));
#22780=CARTESIAN_POINT('Origin',(-0.675,0.,3.605));
#22781=CARTESIAN_POINT('',(-0.675,0.203469899493758,2.275));
#22782=CARTESIAN_POINT('Origin',(-1.0025,0.,3.4));
#22783=CARTESIAN_POINT('',(-1.3,-2.51052593825207E-17,3.195));
#22784=CARTESIAN_POINT('',(-1.0025,-2.51052593825207E-17,3.195));
#22785=CARTESIAN_POINT('',(-1.28373478569368,-0.205,3.4));
#22786=CARTESIAN_POINT('Ctrl Pts',(-1.28373478569368,-0.205,3.4));
#22787=CARTESIAN_POINT('Ctrl Pts',(-1.28373478569368,-0.205,3.37421317147824));
#22788=CARTESIAN_POINT('Ctrl Pts',(-1.28459209201807,-0.199837668299145,
3.34673749165582));
#22789=CARTESIAN_POINT('Ctrl Pts',(-1.2876744550022,-0.178903418830812,
3.29624279964613));
#22790=CARTESIAN_POINT('Ctrl Pts',(-1.28985344916615,-0.163133809500307,
3.27322002921382));
#22791=CARTESIAN_POINT('Ctrl Pts',(-1.29393248914849,-0.12678035877662,
3.23686657849014));
#22792=CARTESIAN_POINT('Ctrl Pts',(-1.29609960028466,-0.103757421316811,
3.22109666480255));
#22793=CARTESIAN_POINT('Ctrl Pts',(-1.29915469398922,-0.0532621572488602,
3.20016219411682));
#22794=CARTESIAN_POINT('Ctrl Pts',(-1.3,-0.0257862780960919,3.195));
#22795=CARTESIAN_POINT('Ctrl Pts',(-1.3,-1.73472347597681E-17,3.195));
#22796=CARTESIAN_POINT('',(-1.3,-5.18464663289491E-17,3.605));
#22797=CARTESIAN_POINT('Ctrl Pts',(-1.3,5.55111512312578E-17,3.605));
#22798=CARTESIAN_POINT('Ctrl Pts',(-1.3,-0.0257862780960919,3.605));
#22799=CARTESIAN_POINT('Ctrl Pts',(-1.29915469398922,-0.0532621572488602,
3.59983780588318));
#22800=CARTESIAN_POINT('Ctrl Pts',(-1.29609960028466,-0.103757421316811,
3.57890333519745));
#22801=CARTESIAN_POINT('Ctrl Pts',(-1.29393248914849,-0.12678035877662,
3.56313342150986));
#22802=CARTESIAN_POINT('Ctrl Pts',(-1.28985344916615,-0.163133809500307,
3.52677997078618));
#22803=CARTESIAN_POINT('Ctrl Pts',(-1.2876744550022,-0.178903418830812,
3.50375720035387));
#22804=CARTESIAN_POINT('Ctrl Pts',(-1.28459209201807,-0.199837668299145,
3.45326250834418));
#22805=CARTESIAN_POINT('Ctrl Pts',(-1.28373478569368,-0.205,3.42578682852176));
#22806=CARTESIAN_POINT('Ctrl Pts',(-1.28373478569368,-0.205,3.4));
#22807=CARTESIAN_POINT('Ctrl Pts',(-1.3,-2.77555756156289E-17,3.195));
#22808=CARTESIAN_POINT('Ctrl Pts',(-1.3,0.0257862780960919,3.195));
#22809=CARTESIAN_POINT('Ctrl Pts',(-1.29915469398922,0.0532621572488602,
3.20016219411682));
#22810=CARTESIAN_POINT('Ctrl Pts',(-1.29609960028466,0.103757421316811,
3.22109666480255));
#22811=CARTESIAN_POINT('Ctrl Pts',(-1.29393248914849,0.12678035877662,3.23686657849014));
#22812=CARTESIAN_POINT('Ctrl Pts',(-1.28985344916615,0.163133809500307,
3.27322002921382));
#22813=CARTESIAN_POINT('Ctrl Pts',(-1.2876744550022,0.178903418830812,3.29624279964613));
#22814=CARTESIAN_POINT('Ctrl Pts',(-1.28459209201807,0.199837668299145,
3.34673749165582));
#22815=CARTESIAN_POINT('Ctrl Pts',(-1.28373478569368,0.205,3.37421317147824));
#22816=CARTESIAN_POINT('Ctrl Pts',(-1.28373478569368,0.205,3.42578682852176));
#22817=CARTESIAN_POINT('Ctrl Pts',(-1.28459209201807,0.199837668299145,
3.45326250834418));
#22818=CARTESIAN_POINT('Ctrl Pts',(-1.2876744550022,0.178903418830812,3.50375720035387));
#22819=CARTESIAN_POINT('Ctrl Pts',(-1.28985344916615,0.163133809500307,
3.52677997078618));
#22820=CARTESIAN_POINT('Ctrl Pts',(-1.29393248914849,0.12678035877662,3.56313342150986));
#22821=CARTESIAN_POINT('Ctrl Pts',(-1.29609960028466,0.103757421316811,
3.57890333519745));
#22822=CARTESIAN_POINT('Ctrl Pts',(-1.29915469398922,0.0532621572488602,
3.59983780588318));
#22823=CARTESIAN_POINT('Ctrl Pts',(-1.3,0.025786278096092,3.605));
#22824=CARTESIAN_POINT('Ctrl Pts',(-1.3,1.17961196366423E-16,3.605));
#22825=CARTESIAN_POINT('Origin',(0.,-0.675,3.4));
#22826=CARTESIAN_POINT('',(0.203469899493758,-0.675,3.375));
#22827=CARTESIAN_POINT('',(0.203469899493758,-0.675,3.425));
#22828=CARTESIAN_POINT('',(0.203469899493758,-0.675,2.275));
#22829=CARTESIAN_POINT('Origin',(0.,-0.675,3.4));
#22830=CARTESIAN_POINT('Origin',(0.,-1.0025,3.4));
#22831=CARTESIAN_POINT('',(-2.29609705471212E-17,-0.705,3.195));
#22832=CARTESIAN_POINT('',(-2.51052593825207E-17,-1.0025,3.195));
#22833=CARTESIAN_POINT('',(-0.203469899493758,-0.675,3.375));
#22834=CARTESIAN_POINT('Ctrl Pts',(-0.203469899493758,-0.675,3.375));
#22835=CARTESIAN_POINT('Ctrl Pts',(-0.201242091014444,-0.675671543655374,
3.35686832130491));
#22836=CARTESIAN_POINT('Ctrl Pts',(-0.196469587434997,-0.67711148178717,
3.33857557904239));
#22837=CARTESIAN_POINT('Ctrl Pts',(-0.178826374035794,-0.682029730751166,
3.29611284356413));
#22838=CARTESIAN_POINT('Ctrl Pts',(-0.16307623613103,-0.68612968485916,
3.27316245584455));
#22839=CARTESIAN_POINT('Ctrl Pts',(-0.126842282640148,-0.693742502155627,
3.23692850235366));
#22840=CARTESIAN_POINT('Ctrl Pts',(-0.103889959828094,-0.697765433634744,
3.22117468990961));
#22841=CARTESIAN_POINT('Ctrl Pts',(-0.0534241842031802,-0.703431290629093,
3.20020642507842));
#22842=CARTESIAN_POINT('Ctrl Pts',(-0.0258990920208441,-0.705,3.195));
#22843=CARTESIAN_POINT('Ctrl Pts',(-6.93889390390723E-18,-0.705,3.195));
#22844=CARTESIAN_POINT('',(-0.203469899493758,-0.675,3.425));
#22845=CARTESIAN_POINT('Origin',(0.,-0.675,3.4));
#22846=CARTESIAN_POINT('Ctrl Pts',(0.203469899493758,-0.675,3.425));
#22847=CARTESIAN_POINT('Ctrl Pts',(0.201242091014444,-0.675671543655374,
3.44313167869509));
#22848=CARTESIAN_POINT('Ctrl Pts',(0.196469587434997,-0.677111481787171,
3.46142442095761));
#22849=CARTESIAN_POINT('Ctrl Pts',(0.178826374035794,-0.682029730751166,
3.50388715643587));
#22850=CARTESIAN_POINT('Ctrl Pts',(0.16307623613103,-0.68612968485916,3.52683754415545));
#22851=CARTESIAN_POINT('Ctrl Pts',(0.126842282640148,-0.693742502155627,
3.56307149764634));
#22852=CARTESIAN_POINT('Ctrl Pts',(0.103889959828094,-0.697765433634744,
3.57882531009039));
#22853=CARTESIAN_POINT('Ctrl Pts',(0.0534241842031802,-0.703431290629093,
3.59979357492158));
#22854=CARTESIAN_POINT('Ctrl Pts',(0.0258990920208441,-0.705,3.605));
#22855=CARTESIAN_POINT('Ctrl Pts',(-0.025899092020844,-0.705,3.605));
#22856=CARTESIAN_POINT('Ctrl Pts',(-0.0534241842031804,-0.703431290629093,
3.59979357492158));
#22857=CARTESIAN_POINT('Ctrl Pts',(-0.103889959828094,-0.697765433634744,
3.57882531009039));
#22858=CARTESIAN_POINT('Ctrl Pts',(-0.126842282640148,-0.693742502155627,
3.56307149764634));
#22859=CARTESIAN_POINT('Ctrl Pts',(-0.16307623613103,-0.68612968485916,
3.52683754415545));
#22860=CARTESIAN_POINT('Ctrl Pts',(-0.178826374035794,-0.682029730751166,
3.50388715643587));
#22861=CARTESIAN_POINT('Ctrl Pts',(-0.196469587434997,-0.67711148178717,
3.46142442095761));
#22862=CARTESIAN_POINT('Ctrl Pts',(-0.201242091014444,-0.675671543655374,
3.44313167869509));
#22863=CARTESIAN_POINT('Ctrl Pts',(-0.203469899493758,-0.675,3.425));
#22864=CARTESIAN_POINT('Ctrl Pts',(-2.08166817117217E-17,-0.705,3.195));
#22865=CARTESIAN_POINT('Ctrl Pts',(0.025899092020844,-0.705,3.195));
#22866=CARTESIAN_POINT('Ctrl Pts',(0.0534241842031803,-0.703431290629093,
3.20020642507842));
#22867=CARTESIAN_POINT('Ctrl Pts',(0.103889959828094,-0.697765433634744,
3.22117468990961));
#22868=CARTESIAN_POINT('Ctrl Pts',(0.126842282640148,-0.693742502155627,
3.23692850235366));
#22869=CARTESIAN_POINT('Ctrl Pts',(0.16307623613103,-0.68612968485916,3.27316245584455));
#22870=CARTESIAN_POINT('Ctrl Pts',(0.178826374035794,-0.682029730751166,
3.29611284356413));
#22871=CARTESIAN_POINT('Ctrl Pts',(0.196469587434997,-0.677111481787171,
3.33857557904239));
#22872=CARTESIAN_POINT('Ctrl Pts',(0.201242091014444,-0.675671543655374,
3.35686832130491));
#22873=CARTESIAN_POINT('Ctrl Pts',(0.203469899493758,-0.675,3.375));
#22874=CARTESIAN_POINT('Origin',(0.,-0.675,3.4));
#22875=CARTESIAN_POINT('',(-0.203469899493758,-0.675,2.275));
#22876=CARTESIAN_POINT('Origin',(0.95,0.,0.4));
#22877=CARTESIAN_POINT('',(-0.95,-1.16341445918999E-16,0.4));
#22878=CARTESIAN_POINT('Origin',(0.,0.,0.4));
#22879=CARTESIAN_POINT('Origin',(0.,0.,0.425));
#22880=CARTESIAN_POINT('',(-1.,-1.22464679914735E-16,0.45));
#22881=CARTESIAN_POINT('Origin',(0.,0.,0.45));
#22882=CARTESIAN_POINT('',(-0.975,-1.19403062916867E-16,0.425));
#22883=CARTESIAN_POINT('Origin',(0.,0.,1.625));
#22884=CARTESIAN_POINT('',(-1.,-1.22464679914735E-16,2.8));
#22885=CARTESIAN_POINT('Origin',(0.,0.,2.8));
#22886=CARTESIAN_POINT('',(-1.,-1.22464679914735E-16,1.625));
#22887=CARTESIAN_POINT('Origin',(1.25,0.,2.8));
#22888=CARTESIAN_POINT('',(-1.25,-1.53080849893419E-16,2.8));
#22889=CARTESIAN_POINT('Origin',(0.,0.,2.8));
#22890=CARTESIAN_POINT('Origin',(0.,0.,2.825));
#22891=CARTESIAN_POINT('',(-1.3,-1.59204083889156E-16,2.85));
#22892=CARTESIAN_POINT('Origin',(0.,0.,2.85));
#22893=CARTESIAN_POINT('',(-1.275,-1.56142466891288E-16,2.825));
#22894=CARTESIAN_POINT('Origin',(0.,0.,3.395));
#22895=CARTESIAN_POINT('',(-1.3,-1.59204083889156E-16,3.94));
#22896=CARTESIAN_POINT('Origin',(0.,0.,3.94));
#22897=CARTESIAN_POINT('',(-1.3,-1.59204083889156E-16,3.395));
#22898=CARTESIAN_POINT('',(-1.3,-1.59204083889156E-16,3.395));
#22899=CARTESIAN_POINT('Origin',(0.,0.,3.97));
#22900=CARTESIAN_POINT('',(-1.24,-1.51856203094272E-16,4.));
#22901=CARTESIAN_POINT('Origin',(0.,0.,4.));
#22902=CARTESIAN_POINT('',(-1.27,-1.55530143491714E-16,3.97));
#22903=CARTESIAN_POINT('Origin',(0.755,0.,4.));
#22904=CARTESIAN_POINT('',(-0.755,-9.24608333356252E-17,4.));
#22905=CARTESIAN_POINT('Origin',(0.,0.,4.));
#22906=CARTESIAN_POINT('Origin',(0.,0.,3.975));
#22907=CARTESIAN_POINT('',(-0.705,-8.63375993398884E-17,3.95));
#22908=CARTESIAN_POINT('',(-0.73,-8.93992163377568E-17,3.975));
#22909=CARTESIAN_POINT('Origin',(0.,0.,3.95));
#22910=CARTESIAN_POINT('Origin',(0.,0.,2.275));
#22911=CARTESIAN_POINT('',(-0.705,-8.63375993398884E-17,2.275));
#22912=CARTESIAN_POINT('',(-0.705,-8.63375993398884E-17,0.6));
#22913=CARTESIAN_POINT('',(-0.705,-8.63375993398884E-17,2.275));
#22914=CARTESIAN_POINT('Origin',(0.,0.,0.6));
#22915=CARTESIAN_POINT('Origin',(0.,0.,0.6));
#38582=UNCERTAINTY_MEASURE_WITH_UNIT(LENGTH_MEASURE(0.001),#38612,
'DISTANCE_ACCURACY_VALUE',
'Maximum model space distance between geometric entities at asserted c
onnectivities');
#38595=UNCERTAINTY_MEASURE_WITH_UNIT(LENGTH_MEASURE(0.001),#38612,
'DISTANCE_ACCURACY_VALUE',
'Maximum model space distance between geometric entities at asserted c
onnectivities');
#38598=(
GEOMETRIC_REPRESENTATION_CONTEXT(3)
GLOBAL_UNCERTAINTY_ASSIGNED_CONTEXT((#38582))
GLOBAL_UNIT_ASSIGNED_CONTEXT((#38612,#38614,#38615))
REPRESENTATION_CONTEXT('','3D')
);
#38611=(
GEOMETRIC_REPRESENTATION_CONTEXT(3)
GLOBAL_UNCERTAINTY_ASSIGNED_CONTEXT((#38595))
GLOBAL_UNIT_ASSIGNED_CONTEXT((#38612,#38614,#38615))
REPRESENTATION_CONTEXT('','3D')
);
#38612=(
LENGTH_UNIT()
NAMED_UNIT(*)
SI_UNIT(.CENTI.,.METRE.)
);
#38614=(
NAMED_UNIT(*)
PLANE_ANGLE_UNIT()
SI_UNIT($,.RADIAN.)
);
#38615=(
NAMED_UNIT(*)
SI_UNIT($,.STERADIAN.)
SOLID_ANGLE_UNIT()
);
#38618=SHAPE_DEFINITION_REPRESENTATION(#38633,#38669);
#38633=PRODUCT_DEFINITION_SHAPE('',$,#38685);
#38669=SHAPE_REPRESENTATION('',(#16581),#38598);
#38682=PRODUCT_DEFINITION_CONTEXT('part definition',#38729,'design');
#38685=PRODUCT_DEFINITION('2026-10-19-02-31-27-829',
'02_Outer_Post_Tube_D20_with_Lock_Collar',#38700,#38682);
#38700=PRODUCT_DEFINITION_FORMATION('',$,#38733);
#38729=APPLICATION_CONTEXT(
'Core Data for Automotive Mechanical Design Process');
#38730=PRODUCT_CONTEXT('part definition',#38729,'mechanical');
#38733=PRODUCT('2026-10-19-02-31-27-829',
'02_Outer_Post_Tube_D20_with_Lock_Collar',$,(#38730));
#38865=COLOUR_RGB('Sky Blue',0.24,0.69,0.87);
#38866=FILL_AREA_STYLE_COLOUR('',#38865);
#38867=FILL_AREA_STYLE('',(#38866));
#38868=SURFACE_STYLE_FILL_AREA(#38867);
#38869=SURFACE_SIDE_STYLE('',(#38868));
#38870=SURFACE_STYLE_USAGE(.BOTH.,#38869);
#38871=PRESENTATION_STYLE_ASSIGNMENT((#38870));
ENDSEC;
END-ISO-10303-21;
